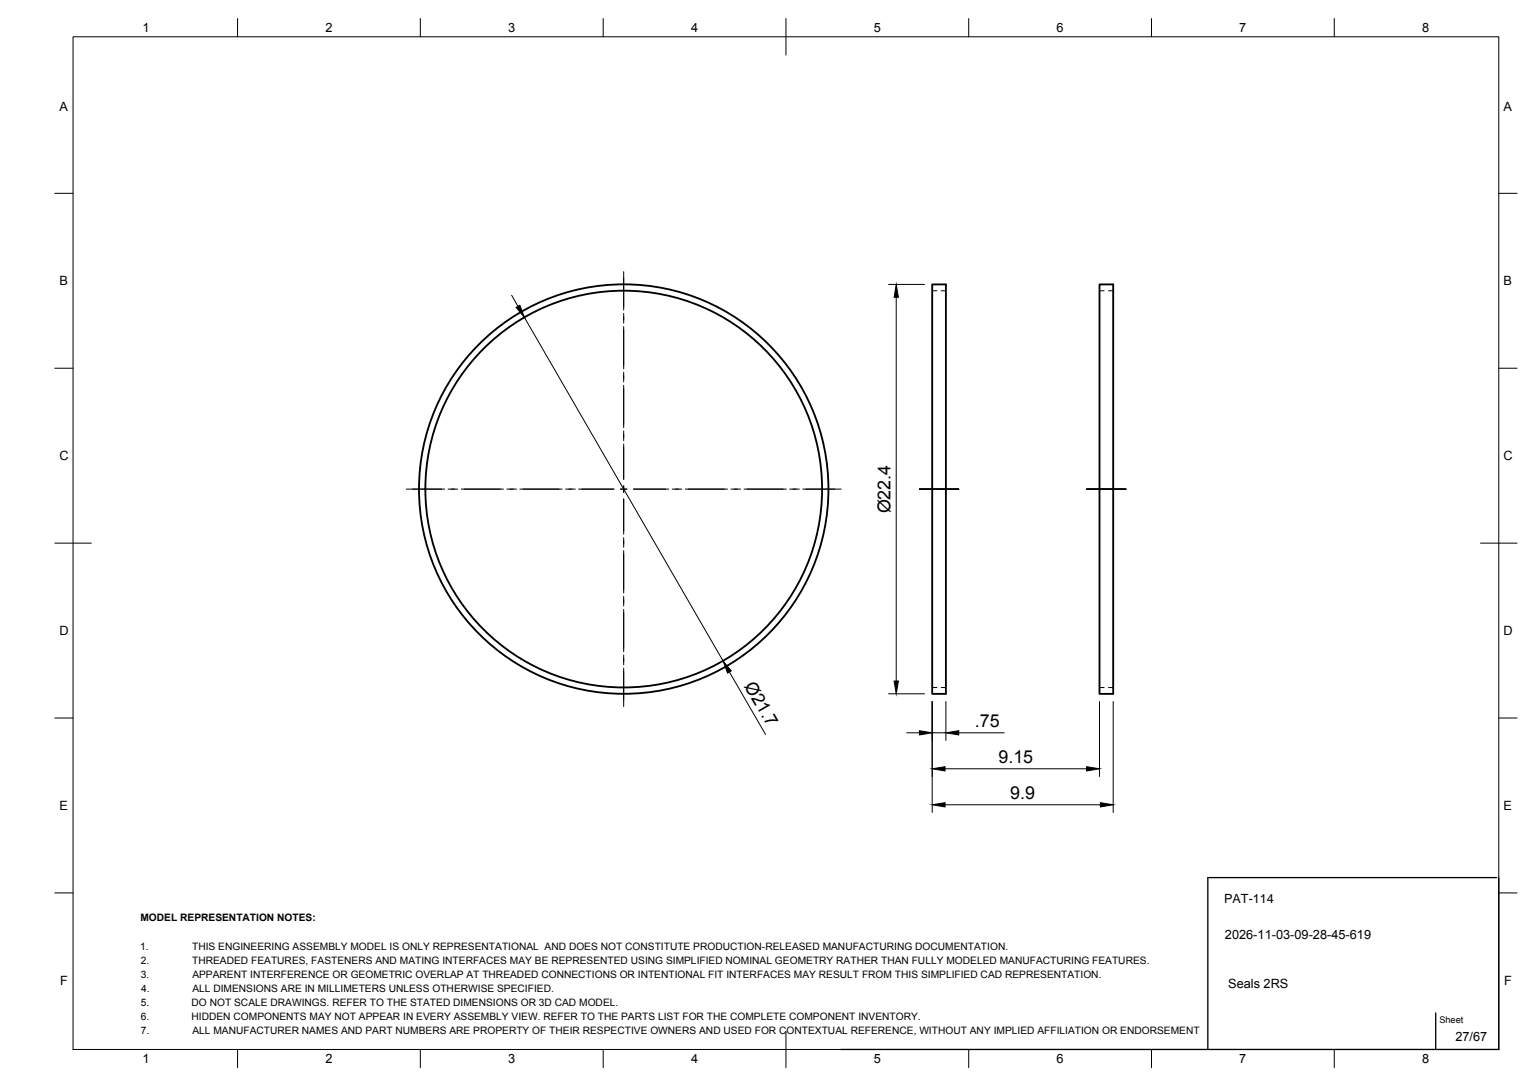
ISO-10303-21;
HEADER;
/* Generated by software containing ST-Developer
 * from STEP Tools, Inc. (www.steptools.com) 
 */

FILE_DESCRIPTION(
/* description */ ('Two-stage gear reducer in split housing'),
/* implementation_level */ '2;1');

FILE_NAME(
/* name */ 'Seals 2RS.step',
/* time_stamp */ '2026-10-28T03:22:31-07:00',
/* author */ (''),
/* organization */ (''),
/* preprocessor_version */ 'ST-DEVELOPER v20.2',
/* originating_system */ 'Autodesk Translation Framework v15.17.0.0',
/* authorisation */ '');

FILE_SCHEMA (('AUTOMOTIVE_DESIGN { 1 0 10303 214 3 1 1 }'));
ENDSEC;

DATA;
#10=MECHANICAL_DESIGN_GEOMETRIC_PRESENTATION_REPRESENTATION('',(#1261,#1262),#73366);
#1143=SHAPE_REPRESENTATION_RELATIONSHIP('SRR','None',#73631,#1199);
#1199=ADVANCED_BREP_SHAPE_REPRESENTATION('',(#1331,#1332),#73327);
#1261=STYLED_ITEM('',(#73988),#1331);
#1262=STYLED_ITEM('',(#73988),#1332);
#1331=MANIFOLD_SOLID_BREP('Body1',#16150);
#1332=MANIFOLD_SOLID_BREP('Body2',#16151);
#1524=FACE_BOUND('',#3404,.T.);
#1525=FACE_BOUND('',#3407,.T.);
#1526=FACE_BOUND('',#3410,.T.);
#1527=FACE_BOUND('',#3413,.T.);
#1767=PLANE('',#17523);
#1768=PLANE('',#17528);
#1769=PLANE('',#17531);
#1770=PLANE('',#17536);
#2340=FACE_OUTER_BOUND('',#3403,.T.);
#2341=FACE_OUTER_BOUND('',#3405,.T.);
#2342=FACE_OUTER_BOUND('',#3406,.T.);
#2343=FACE_OUTER_BOUND('',#3408,.T.);
#2344=FACE_OUTER_BOUND('',#3409,.T.);
#2345=FACE_OUTER_BOUND('',#3411,.T.);
#2346=FACE_OUTER_BOUND('',#3412,.T.);
#2347=FACE_OUTER_BOUND('',#3414,.T.);
#3403=EDGE_LOOP('',(#11989));
#3404=EDGE_LOOP('',(#11990));
#3405=EDGE_LOOP('',(#11991,#11992,#11993,#11994));
#3406=EDGE_LOOP('',(#11995));
#3407=EDGE_LOOP('',(#11996));
#3408=EDGE_LOOP('',(#11997,#11998,#11999,#12000));
#3409=EDGE_LOOP('',(#12001));
#3410=EDGE_LOOP('',(#12002));
#3411=EDGE_LOOP('',(#12003,#12004,#12005,#12006));
#3412=EDGE_LOOP('',(#12007));
#3413=EDGE_LOOP('',(#12008));
#3414=EDGE_LOOP('',(#12009,#12010,#12011,#12012));
#4435=LINE('',#24681,#5459);
#4436=LINE('',#24686,#5460);
#4437=LINE('',#24695,#5461);
#4438=LINE('',#24700,#5462);
#5459=VECTOR('',#20269,1.119765);
#5460=VECTOR('',#20276,1.085235);
#5461=VECTOR('',#20287,1.119765);
#5462=VECTOR('',#20294,1.085235);
#6452=CIRCLE('',#17524,1.119765);
#6453=CIRCLE('',#17525,1.085235);
#6454=CIRCLE('',#17527,1.119765);
#6455=CIRCLE('',#17529,1.085235);
#6456=CIRCLE('',#17532,1.119765);
#6457=CIRCLE('',#17533,1.085235);
#6458=CIRCLE('',#17535,1.119765);
#6459=CIRCLE('',#17537,1.085235);
#7325=VERTEX_POINT('',#24674);
#7326=VERTEX_POINT('',#24676);
#7327=VERTEX_POINT('',#24679);
#7328=VERTEX_POINT('',#24683);
#7329=VERTEX_POINT('',#24688);
#7330=VERTEX_POINT('',#24690);
#7331=VERTEX_POINT('',#24693);
#7332=VERTEX_POINT('',#24697);
#9048=EDGE_CURVE('',#7325,#7325,#6452,.T.);
#9049=EDGE_CURVE('',#7326,#7326,#6453,.T.);
#9050=EDGE_CURVE('',#7327,#7327,#6454,.T.);
#9051=EDGE_CURVE('',#7327,#7325,#4435,.T.);
#9052=EDGE_CURVE('',#7328,#7328,#6455,.T.);
#9053=EDGE_CURVE('',#7328,#7326,#4436,.T.);
#9054=EDGE_CURVE('',#7329,#7329,#6456,.T.);
#9055=EDGE_CURVE('',#7330,#7330,#6457,.T.);
#9056=EDGE_CURVE('',#7331,#7331,#6458,.T.);
#9057=EDGE_CURVE('',#7331,#7329,#4437,.T.);
#9058=EDGE_CURVE('',#7332,#7332,#6459,.T.);
#9059=EDGE_CURVE('',#7332,#7330,#4438,.T.);
#11989=ORIENTED_EDGE('',*,*,#9048,.F.);
#11990=ORIENTED_EDGE('',*,*,#9049,.T.);
#11991=ORIENTED_EDGE('',*,*,#9050,.F.);
#11992=ORIENTED_EDGE('',*,*,#9051,.T.);
#11993=ORIENTED_EDGE('',*,*,#9048,.T.);
#11994=ORIENTED_EDGE('',*,*,#9051,.F.);
#11995=ORIENTED_EDGE('',*,*,#9050,.T.);
#11996=ORIENTED_EDGE('',*,*,#9052,.F.);
#11997=ORIENTED_EDGE('',*,*,#9052,.T.);
#11998=ORIENTED_EDGE('',*,*,#9053,.T.);
#11999=ORIENTED_EDGE('',*,*,#9049,.F.);
#12000=ORIENTED_EDGE('',*,*,#9053,.F.);
#12001=ORIENTED_EDGE('',*,*,#9054,.F.);
#12002=ORIENTED_EDGE('',*,*,#9055,.T.);
#12003=ORIENTED_EDGE('',*,*,#9056,.F.);
#12004=ORIENTED_EDGE('',*,*,#9057,.T.);
#12005=ORIENTED_EDGE('',*,*,#9054,.T.);
#12006=ORIENTED_EDGE('',*,*,#9057,.F.);
#12007=ORIENTED_EDGE('',*,*,#9056,.T.);
#12008=ORIENTED_EDGE('',*,*,#9058,.F.);
#12009=ORIENTED_EDGE('',*,*,#9058,.T.);
#12010=ORIENTED_EDGE('',*,*,#9059,.T.);
#12011=ORIENTED_EDGE('',*,*,#9055,.F.);
#12012=ORIENTED_EDGE('',*,*,#9059,.F.);
#15057=CYLINDRICAL_SURFACE('',#17526,1.119765);
#15058=CYLINDRICAL_SURFACE('',#17530,1.085235);
#15059=CYLINDRICAL_SURFACE('',#17534,1.119765);
#15060=CYLINDRICAL_SURFACE('',#17538,1.085235);
#15547=ADVANCED_FACE('',(#2340,#1524),#1767,.T.);
#15548=ADVANCED_FACE('',(#2341),#15057,.T.);
#15549=ADVANCED_FACE('',(#2342,#1525),#1768,.T.);
#15550=ADVANCED_FACE('',(#2343),#15058,.F.);
#15551=ADVANCED_FACE('',(#2344,#1526),#1769,.T.);
#15552=ADVANCED_FACE('',(#2345),#15059,.T.);
#15553=ADVANCED_FACE('',(#2346,#1527),#1770,.T.);
#15554=ADVANCED_FACE('',(#2347),#15060,.F.);
#16150=CLOSED_SHELL('',(#15547,#15548,#15549,#15550));
#16151=CLOSED_SHELL('',(#15551,#15552,#15553,#15554));
#17522=AXIS2_PLACEMENT_3D('',#24672,#20257,#20258);
#17523=AXIS2_PLACEMENT_3D('',#24673,#20259,#20260);
#17524=AXIS2_PLACEMENT_3D('',#24675,#20261,#20262);
#17525=AXIS2_PLACEMENT_3D('',#24677,#20263,#20264);
#17526=AXIS2_PLACEMENT_3D('',#24678,#20265,#20266);
#17527=AXIS2_PLACEMENT_3D('',#24680,#20267,#20268);
#17528=AXIS2_PLACEMENT_3D('',#24682,#20270,#20271);
#17529=AXIS2_PLACEMENT_3D('',#24684,#20272,#20273);
#17530=AXIS2_PLACEMENT_3D('',#24685,#20274,#20275);
#17531=AXIS2_PLACEMENT_3D('',#24687,#20277,#20278);
#17532=AXIS2_PLACEMENT_3D('',#24689,#20279,#20280);
#17533=AXIS2_PLACEMENT_3D('',#24691,#20281,#20282);
#17534=AXIS2_PLACEMENT_3D('',#24692,#20283,#20284);
#17535=AXIS2_PLACEMENT_3D('',#24694,#20285,#20286);
#17536=AXIS2_PLACEMENT_3D('',#24696,#20288,#20289);
#17537=AXIS2_PLACEMENT_3D('',#24698,#20290,#20291);
#17538=AXIS2_PLACEMENT_3D('',#24699,#20292,#20293);
#20257=DIRECTION('axis',(0.,0.,1.));
#20258=DIRECTION('refdir',(1.,0.,0.));
#20259=DIRECTION('center_axis',(0.,1.,0.));
#20260=DIRECTION('ref_axis',(0.,0.,1.));
#20261=DIRECTION('center_axis',(0.,-1.,0.));
#20262=DIRECTION('ref_axis',(1.,0.,0.));
#20263=DIRECTION('center_axis',(0.,-1.,0.));
#20264=DIRECTION('ref_axis',(1.,0.,0.));
#20265=DIRECTION('center_axis',(0.,-1.,0.));
#20266=DIRECTION('ref_axis',(1.,0.,0.));
#20267=DIRECTION('center_axis',(0.,-1.,0.));
#20268=DIRECTION('ref_axis',(1.,0.,0.));
#20269=DIRECTION('',(0.,1.,0.));
#20270=DIRECTION('center_axis',(0.,-1.,0.));
#20271=DIRECTION('ref_axis',(0.,0.,-1.));
#20272=DIRECTION('center_axis',(0.,-1.,0.));
#20273=DIRECTION('ref_axis',(1.,0.,0.));
#20274=DIRECTION('center_axis',(0.,-1.,0.));
#20275=DIRECTION('ref_axis',(1.,0.,0.));
#20276=DIRECTION('',(0.,1.,0.));
#20277=DIRECTION('center_axis',(0.,1.,0.));
#20278=DIRECTION('ref_axis',(0.,0.,1.));
#20279=DIRECTION('center_axis',(0.,-1.,0.));
#20280=DIRECTION('ref_axis',(1.,0.,0.));
#20281=DIRECTION('center_axis',(0.,-1.,0.));
#20282=DIRECTION('ref_axis',(1.,0.,0.));
#20283=DIRECTION('center_axis',(0.,-1.,0.));
#20284=DIRECTION('ref_axis',(1.,0.,0.));
#20285=DIRECTION('center_axis',(0.,-1.,0.));
#20286=DIRECTION('ref_axis',(1.,0.,0.));
#20287=DIRECTION('',(0.,1.,0.));
#20288=DIRECTION('center_axis',(0.,-1.,0.));
#20289=DIRECTION('ref_axis',(0.,0.,-1.));
#20290=DIRECTION('center_axis',(0.,-1.,0.));
#20291=DIRECTION('ref_axis',(1.,0.,0.));
#20292=DIRECTION('center_axis',(0.,-1.,0.));
#20293=DIRECTION('ref_axis',(1.,0.,0.));
#20294=DIRECTION('',(0.,1.,0.));
#24672=CARTESIAN_POINT('',(0.,0.,0.));
#24673=CARTESIAN_POINT('Origin',(1.119765,0.495,0.));
#24674=CARTESIAN_POINT('',(-1.119765,0.495,-1.37131662304724E-16));
#24675=CARTESIAN_POINT('Origin',(0.,0.495,0.));
#24676=CARTESIAN_POINT('',(-1.085235,0.495,-1.32902956907268E-16));
#24677=CARTESIAN_POINT('Origin',(0.,0.495,0.));
#24678=CARTESIAN_POINT('Origin',(0.,0.4575,0.));
#24679=CARTESIAN_POINT('',(-1.119765,0.42,-1.37131662304724E-16));
#24680=CARTESIAN_POINT('Origin',(0.,0.42,0.));
#24681=CARTESIAN_POINT('',(-1.119765,0.4575,-1.37131662304724E-16));
#24682=CARTESIAN_POINT('Origin',(1.085235,0.42,0.));
#24683=CARTESIAN_POINT('',(-1.085235,0.42,-1.32902956907268E-16));
#24684=CARTESIAN_POINT('Origin',(0.,0.42,0.));
#24685=CARTESIAN_POINT('Origin',(0.,0.4575,0.));
#24686=CARTESIAN_POINT('',(-1.085235,0.4575,-1.32902956907268E-16));
#24687=CARTESIAN_POINT('Origin',(1.119765,-0.42,0.));
#24688=CARTESIAN_POINT('',(-1.119765,-0.42,-1.37131662304724E-16));
#24689=CARTESIAN_POINT('Origin',(0.,-0.42,0.));
#24690=CARTESIAN_POINT('',(-1.085235,-0.42,-1.32902956907268E-16));
#24691=CARTESIAN_POINT('Origin',(0.,-0.42,0.));
#24692=CARTESIAN_POINT('Origin',(0.,-0.4575,0.));
#24693=CARTESIAN_POINT('',(-1.119765,-0.495,-1.37131662304724E-16));
#24694=CARTESIAN_POINT('Origin',(0.,-0.495,0.));
#24695=CARTESIAN_POINT('',(-1.119765,-0.4575,-1.37131662304724E-16));
#24696=CARTESIAN_POINT('Origin',(1.085235,-0.495,0.));
#24697=CARTESIAN_POINT('',(-1.085235,-0.495,-1.32902956907268E-16));
#24698=CARTESIAN_POINT('Origin',(0.,-0.495,0.));
#24699=CARTESIAN_POINT('Origin',(0.,-0.4575,0.));
#24700=CARTESIAN_POINT('',(-1.085235,-0.4575,-1.32902956907268E-16));
#73263=UNCERTAINTY_MEASURE_WITH_UNIT(LENGTH_MEASURE(0.001),#73367,
'DISTANCE_ACCURACY_VALUE',
'Maximum model space distance between geometric entities at asserted c
onnectivities');
#73302=UNCERTAINTY_MEASURE_WITH_UNIT(LENGTH_MEASURE(0.001),#73367,
'DISTANCE_ACCURACY_VALUE',
'Maximum model space distance between geometric entities at asserted c
onnectivities');
#73327=(
GEOMETRIC_REPRESENTATION_CONTEXT(3)
GLOBAL_UNCERTAINTY_ASSIGNED_CONTEXT((#73263))
GLOBAL_UNIT_ASSIGNED_CONTEXT((#73367,#73369,#73370))
REPRESENTATION_CONTEXT('','3D')
);
#73366=(
GEOMETRIC_REPRESENTATION_CONTEXT(3)
GLOBAL_UNCERTAINTY_ASSIGNED_CONTEXT((#73302))
GLOBAL_UNIT_ASSIGNED_CONTEXT((#73367,#73369,#73370))
REPRESENTATION_CONTEXT('','3D')
);
#73367=(
LENGTH_UNIT()
NAMED_UNIT(*)
SI_UNIT(.CENTI.,.METRE.)
);
#73369=(
NAMED_UNIT(*)
PLANE_ANGLE_UNIT()
SI_UNIT($,.RADIAN.)
);
#73370=(
NAMED_UNIT(*)
SI_UNIT($,.STERADIAN.)
SOLID_ANGLE_UNIT()
);
#73395=SHAPE_DEFINITION_REPRESENTATION(#73458,#73631);
#73458=PRODUCT_DEFINITION_SHAPE('',$,#73695);
#73631=SHAPE_REPRESENTATION('',(#17522),#73327);
#73670=PRODUCT_DEFINITION_CONTEXT('part definition',#73861,'design');
#73695=PRODUCT_DEFINITION('Seals 2RS','Seals 2RS',#73758,#73670);
#73758=PRODUCT_DEFINITION_FORMATION('',$,#73887);
#73861=APPLICATION_CONTEXT(
'Core Data for Automotive Mechanical Design Process');
#73862=PRODUCT_CONTEXT('part definition',#73861,'mechanical');
#73887=PRODUCT('Seals 2RS','Seals 2RS','Seals 2RS',(#73862));
#73982=COLOUR_RGB('Grey',0.48,0.52,0.57);
#73983=FILL_AREA_STYLE_COLOUR('',#73982);
#73984=FILL_AREA_STYLE('',(#73983));
#73985=SURFACE_STYLE_FILL_AREA(#73984);
#73986=SURFACE_SIDE_STYLE('',(#73985));
#73987=SURFACE_STYLE_USAGE(.BOTH.,#73986);
#73988=PRESENTATION_STYLE_ASSIGNMENT((#73987));
ENDSEC;
END-ISO-10303-21;
